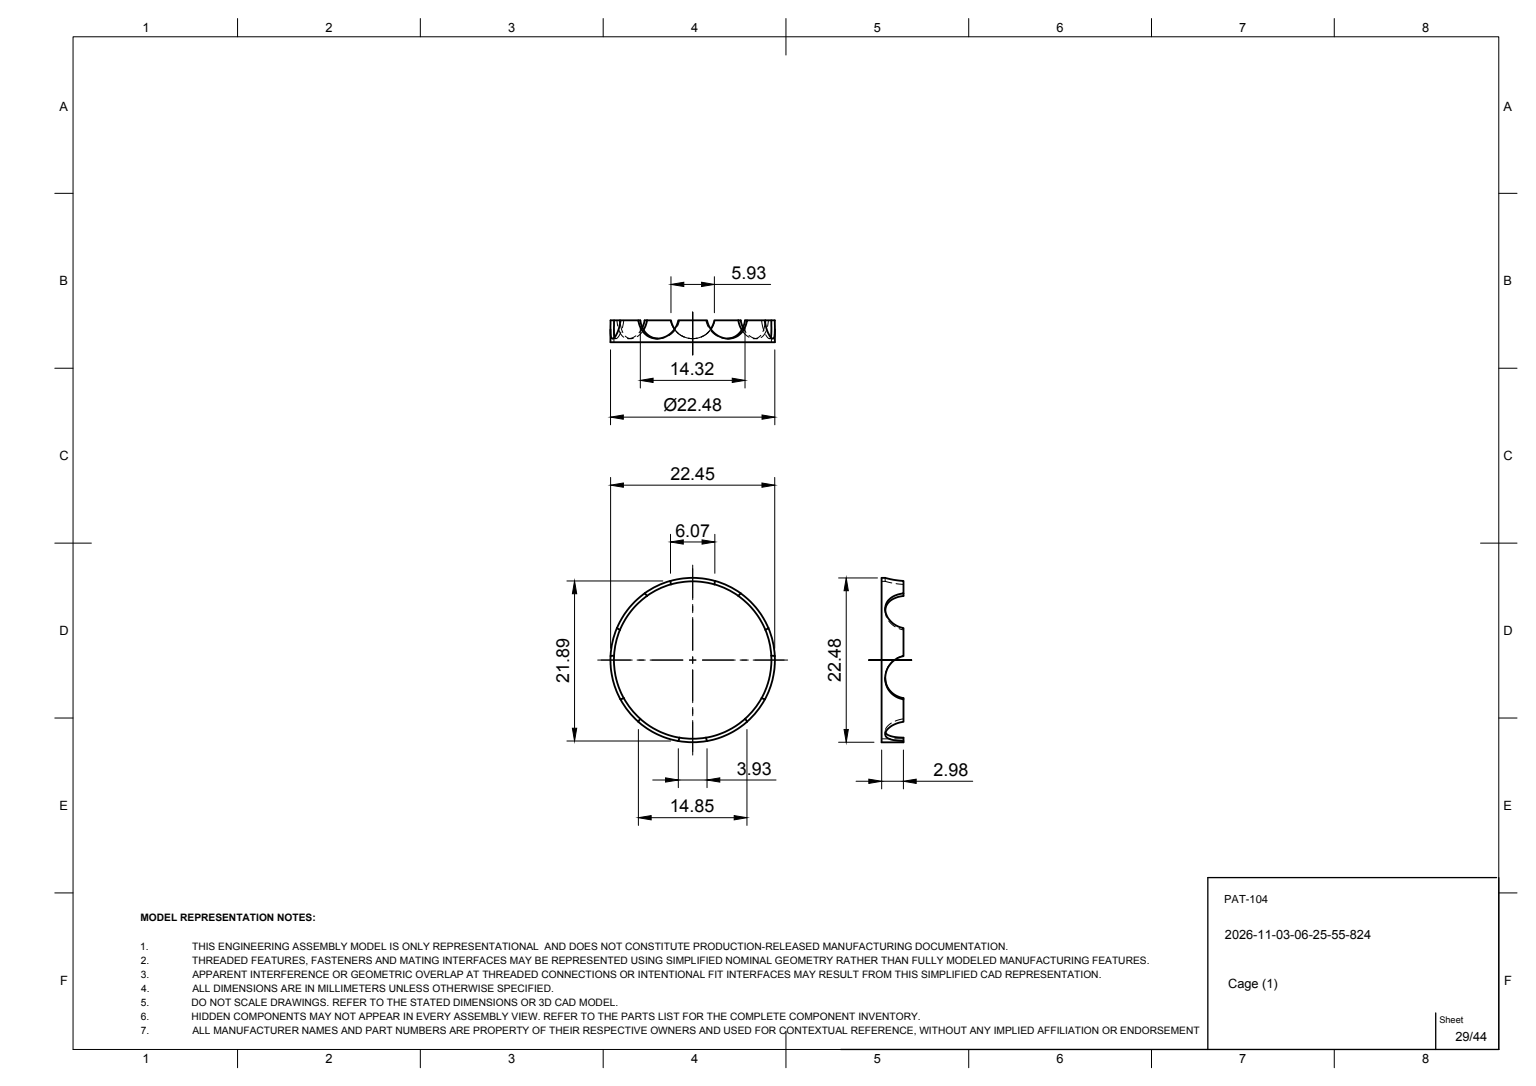
ISO-10303-21;
HEADER;
/* Generated by software containing ST-Developer
 * from STEP Tools, Inc. (www.steptools.com) 
 */

FILE_DESCRIPTION(
/* description */ ('Timing belt drive module 2 mm Pitch Timing 20T-40T'),

/* implementation_level */ '2;1');

FILE_NAME(
/* name */ 'Cage (1).step',
/* time_stamp */ '2026-10-28T03:25:12-07:00',
/* author */ (''),
/* organization */ (''),
/* preprocessor_version */ 'ST-DEVELOPER v20.2',
/* originating_system */ 'Autodesk Translation Framework v15.17.0.0',
/* authorisation */ '');

FILE_SCHEMA (('AUTOMOTIVE_DESIGN { 1 0 10303 214 3 1 1 }'));
ENDSEC;

DATA;
#10=MECHANICAL_DESIGN_GEOMETRIC_PRESENTATION_REPRESENTATION('',(#563),#17830);
#327=B_SPLINE_CURVE_WITH_KNOTS('',3,(#15464,#15465,#15466,#15467,#15468,
#15469,#15470,#15471,#15472,#15473,#15474,#15475,#15476,#15477,#15478,#15479,
#15480,#15481,#15482,#15483,#15484,#15485),.UNSPECIFIED.,.F.,.F.,(4,2,2,
2,2,2,2,2,2,2,4),(0.0591825211272536,0.157966726598481,0.236950089897721,
0.315933453196962,0.391576304923761,0.46721915665056,0.54286200837736,0.618504860104159,
0.697488223403399,0.77647158670264,0.875255792173867),.UNSPECIFIED.);
#328=B_SPLINE_CURVE_WITH_KNOTS('',3,(#15489,#15490,#15491,#15492,#15493,
#15494,#15495,#15496,#15497,#15498,#15499,#15500,#15501,#15502,#15503,#15504,
#15505,#15506,#15507,#15508,#15509,#15510),.UNSPECIFIED.,.F.,.F.,(4,2,2,
2,2,2,2,2,2,2,4),(0.0581119756758434,0.106553146291161,0.213106292582322,
0.30849933801665,0.386091982889075,0.4636846277615,0.541277272633925,0.61886991750635,
0.714262962940678,0.820816109231839,0.869257279847157),.UNSPECIFIED.);
#329=B_SPLINE_CURVE_WITH_KNOTS('',3,(#15516,#15517,#15518,#15519,#15520,
#15521,#15522,#15523,#15524,#15525,#15526,#15527,#15528,#15529,#15530,#15531,
#15532,#15533,#15534,#15535,#15536,#15537),.UNSPECIFIED.,.F.,.F.,(4,2,2,
2,2,2,2,2,2,2,4),(0.0581119756758434,0.106553146291161,0.213106292582322,
0.30849933801665,0.386091982889075,0.4636846277615,0.541277272633925,0.61886991750635,
0.714262962940679,0.820816109231839,0.869257279847157),.UNSPECIFIED.);
#330=B_SPLINE_CURVE_WITH_KNOTS('',3,(#15541,#15542,#15543,#15544,#15545,
#15546,#15547,#15548,#15549,#15550,#15551,#15552,#15553,#15554,#15555,#15556,
#15557,#15558,#15559,#15560,#15561,#15562),.UNSPECIFIED.,.F.,.F.,(4,2,2,
2,2,2,2,2,2,2,4),(0.0581119756758433,0.106553146291161,0.213106292582322,
0.308499338016649,0.386091982889075,0.4636846277615,0.541277272633925,0.61886991750635,
0.714262962940678,0.820816109231839,0.869257279847157),.UNSPECIFIED.);
#331=B_SPLINE_CURVE_WITH_KNOTS('',3,(#15571,#15572,#15573,#15574,#15575,
#15576,#15577,#15578,#15579,#15580,#15581,#15582,#15583,#15584,#15585,#15586,
#15587,#15588,#15589,#15590,#15591,#15592),.UNSPECIFIED.,.F.,.F.,(4,2,2,
2,2,2,2,2,2,2,4),(0.0581119756758433,0.106553146291161,0.213106292582322,
0.30849933801665,0.386091982889075,0.4636846277615,0.541277272633925,0.61886991750635,
0.714262962940678,0.820816109231839,0.869257279847157),.UNSPECIFIED.);
#332=B_SPLINE_CURVE_WITH_KNOTS('',3,(#15596,#15597,#15598,#15599,#15600,
#15601,#15602,#15603,#15604,#15605,#15606,#15607,#15608,#15609,#15610,#15611,
#15612,#15613,#15614,#15615,#15616,#15617),.UNSPECIFIED.,.F.,.F.,(4,2,2,
2,2,2,2,2,2,2,4),(0.0581119756758434,0.106553146291161,0.213106292582322,
0.30849933801665,0.386091982889075,0.4636846277615,0.541277272633925,0.61886991750635,
0.714262962940678,0.820816109231839,0.869257279847157),.UNSPECIFIED.);
#333=B_SPLINE_CURVE_WITH_KNOTS('',3,(#15621,#15622,#15623,#15624,#15625,
#15626,#15627,#15628,#15629,#15630,#15631,#15632,#15633,#15634,#15635,#15636,
#15637,#15638,#15639,#15640,#15641,#15642),.UNSPECIFIED.,.F.,.F.,(4,2,2,
2,2,2,2,2,2,2,4),(0.0581119756758434,0.106553146291161,0.213106292582322,
0.30849933801665,0.386091982889075,0.4636846277615,0.541277272633925,0.61886991750635,
0.714262962940678,0.820816109231839,0.869257279847157),.UNSPECIFIED.);
#334=B_SPLINE_CURVE_WITH_KNOTS('',3,(#15646,#15647,#15648,#15649,#15650,
#15651,#15652,#15653,#15654,#15655,#15656,#15657,#15658,#15659,#15660,#15661,
#15662,#15663,#15664,#15665,#15666,#15667),.UNSPECIFIED.,.F.,.F.,(4,2,2,
2,2,2,2,2,2,2,4),(0.0581119756758433,0.106553146291161,0.213106292582322,
0.30849933801665,0.386091982889075,0.4636846277615,0.541277272633925,0.61886991750635,
0.714262962940678,0.820816109231839,0.869257279847157),.UNSPECIFIED.);
#335=B_SPLINE_CURVE_WITH_KNOTS('',3,(#15675,#15676,#15677,#15678,#15679,
#15680,#15681,#15682,#15683,#15684,#15685,#15686,#15687,#15688,#15689,#15690,
#15691,#15692,#15693,#15694,#15695,#15696),.UNSPECIFIED.,.F.,.F.,(4,2,2,
2,2,2,2,2,2,2,4),(0.0591825211272536,0.157966726598481,0.236950089897721,
0.315933453196962,0.391576304923761,0.467219156650561,0.54286200837736,
0.618504860104159,0.697488223403399,0.77647158670264,0.875255792173867),
 .UNSPECIFIED.);
#336=B_SPLINE_CURVE_WITH_KNOTS('',3,(#15704,#15705,#15706,#15707,#15708,
#15709,#15710,#15711,#15712,#15713,#15714,#15715,#15716,#15717,#15718,#15719,
#15720,#15721,#15722,#15723,#15724,#15725),.UNSPECIFIED.,.F.,.F.,(4,2,2,
2,2,2,2,2,2,2,4),(0.0591825211272536,0.157966726598481,0.236950089897722,
0.315933453196962,0.391576304923761,0.467219156650561,0.54286200837736,
0.618504860104159,0.697488223403399,0.77647158670264,0.875255792173867),
 .UNSPECIFIED.);
#337=B_SPLINE_CURVE_WITH_KNOTS('',3,(#15735,#15736,#15737,#15738,#15739,
#15740,#15741,#15742,#15743,#15744,#15745,#15746,#15747,#15748,#15749,#15750,
#15751,#15752,#15753,#15754,#15755,#15756),.UNSPECIFIED.,.F.,.F.,(4,2,2,
2,2,2,2,2,2,2,4),(0.0591825211272536,0.157966726598481,0.236950089897721,
0.315933453196962,0.391576304923761,0.46721915665056,0.54286200837736,0.618504860104159,
0.697488223403399,0.77647158670264,0.875255792173867),.UNSPECIFIED.);
#338=B_SPLINE_CURVE_WITH_KNOTS('',3,(#15764,#15765,#15766,#15767,#15768,
#15769,#15770,#15771,#15772,#15773,#15774,#15775,#15776,#15777,#15778,#15779,
#15780,#15781,#15782,#15783,#15784,#15785),.UNSPECIFIED.,.F.,.F.,(4,2,2,
2,2,2,2,2,2,2,4),(0.0591825211272536,0.157966726598481,0.236950089897721,
0.315933453196962,0.391576304923761,0.46721915665056,0.542862008377359,
0.618504860104159,0.697488223403399,0.776471586702639,0.875255792173867),
 .UNSPECIFIED.);
#339=B_SPLINE_CURVE_WITH_KNOTS('',3,(#15793,#15794,#15795,#15796,#15797,
#15798,#15799,#15800,#15801,#15802,#15803,#15804,#15805,#15806,#15807,#15808,
#15809,#15810,#15811,#15812,#15813,#15814),.UNSPECIFIED.,.F.,.F.,(4,2,2,
2,2,2,2,2,2,2,4),(0.0591825211272536,0.157966726598481,0.236950089897721,
0.315933453196962,0.391576304923761,0.46721915665056,0.54286200837736,0.618504860104159,
0.697488223403399,0.77647158670264,0.875255792173867),.UNSPECIFIED.);
#340=B_SPLINE_CURVE_WITH_KNOTS('',3,(#15823,#15824,#15825,#15826,#15827,
#15828,#15829,#15830,#15831,#15832,#15833,#15834,#15835,#15836,#15837,#15838,
#15839,#15840,#15841,#15842,#15843,#15844),.UNSPECIFIED.,.F.,.F.,(4,2,2,
2,2,2,2,2,2,2,4),(0.0591825211272536,0.157966726598481,0.236950089897721,
0.315933453196962,0.391576304923761,0.46721915665056,0.542862008377359,
0.618504860104159,0.697488223403399,0.776471586702639,0.875255792173867),
 .UNSPECIFIED.);
#408=SPHERICAL_SURFACE('',#10097,0.309556);
#409=SPHERICAL_SURFACE('',#10113,0.309556);
#410=SPHERICAL_SURFACE('',#10118,0.309556);
#411=SPHERICAL_SURFACE('',#10124,0.309556);
#412=SPHERICAL_SURFACE('',#10129,0.309556);
#413=SPHERICAL_SURFACE('',#10134,0.309556);
#414=SPHERICAL_SURFACE('',#10142,0.309556);
#463=SHAPE_REPRESENTATION_RELATIONSHIP('SRR','None',#18035,#506);
#506=ADVANCED_BREP_SHAPE_REPRESENTATION('',(#620),#17810);
#563=STYLED_ITEM('',(#18317),#620);
#620=MANIFOLD_SOLID_BREP('Continuous crown cage',#9021);
#724=FACE_BOUND('',#1845,.T.);
#886=PLANE('',#10110);
#887=PLANE('',#10115);
#888=PLANE('',#10120);
#889=PLANE('',#10126);
#890=PLANE('',#10131);
#891=PLANE('',#10140);
#892=PLANE('',#10144);
#893=PLANE('',#10145);
#1221=FACE_OUTER_BOUND('',#1829,.T.);
#1222=FACE_OUTER_BOUND('',#1830,.T.);
#1223=FACE_OUTER_BOUND('',#1831,.T.);
#1224=FACE_OUTER_BOUND('',#1832,.T.);
#1225=FACE_OUTER_BOUND('',#1833,.T.);
#1226=FACE_OUTER_BOUND('',#1834,.T.);
#1227=FACE_OUTER_BOUND('',#1835,.T.);
#1228=FACE_OUTER_BOUND('',#1836,.T.);
#1229=FACE_OUTER_BOUND('',#1837,.T.);
#1230=FACE_OUTER_BOUND('',#1838,.T.);
#1231=FACE_OUTER_BOUND('',#1839,.T.);
#1232=FACE_OUTER_BOUND('',#1840,.T.);
#1233=FACE_OUTER_BOUND('',#1841,.T.);
#1234=FACE_OUTER_BOUND('',#1842,.T.);
#1235=FACE_OUTER_BOUND('',#1843,.T.);
#1236=FACE_OUTER_BOUND('',#1844,.T.);
#1237=FACE_OUTER_BOUND('',#1846,.T.);
#1829=EDGE_LOOP('',(#6901,#6902,#6903,#6904));
#1830=EDGE_LOOP('',(#6905,#6906,#6907,#6908,#6909,#6910,#6911,#6912,#6913,
#6914,#6915,#6916,#6917,#6918,#6919,#6920,#6921,#6922));
#1831=EDGE_LOOP('',(#6923,#6924,#6925,#6926));
#1832=EDGE_LOOP('',(#6927,#6928,#6929,#6930));
#1833=EDGE_LOOP('',(#6931,#6932,#6933,#6934));
#1834=EDGE_LOOP('',(#6935,#6936,#6937,#6938));
#1835=EDGE_LOOP('',(#6939,#6940,#6941,#6942,#6943,#6944));
#1836=EDGE_LOOP('',(#6945,#6946,#6947,#6948));
#1837=EDGE_LOOP('',(#6949,#6950,#6951,#6952));
#1838=EDGE_LOOP('',(#6953,#6954,#6955,#6956));
#1839=EDGE_LOOP('',(#6957,#6958,#6959,#6960));
#1840=EDGE_LOOP('',(#6961,#6962,#6963,#6964));
#1841=EDGE_LOOP('',(#6965,#6966,#6967,#6968,#6969,#6970,#6971,#6972,#6973,
#6974,#6975,#6976,#6977,#6978,#6979,#6980,#6981,#6982));
#1842=EDGE_LOOP('',(#6983,#6984,#6985,#6986));
#1843=EDGE_LOOP('',(#6987,#6988,#6989,#6990));
#1844=EDGE_LOOP('',(#6991));
#1845=EDGE_LOOP('',(#6992));
#1846=EDGE_LOOP('',(#6993,#6994,#6995,#6996));
#2427=CIRCLE('',#10098,0.303778037777585);
#2428=CIRCLE('',#10099,0.303778037777585);
#2429=CIRCLE('',#10101,1.123812);
#2430=CIRCLE('',#10102,1.123812);
#2431=CIRCLE('',#10103,1.123812);
#2432=CIRCLE('',#10104,1.123812);
#2433=CIRCLE('',#10105,1.123812);
#2434=CIRCLE('',#10106,1.123812);
#2435=CIRCLE('',#10107,1.123812);
#2436=CIRCLE('',#10108,1.123812);
#2437=CIRCLE('',#10109,1.123812);
#2438=CIRCLE('',#10111,1.076188);
#2439=CIRCLE('',#10112,0.303778037777585);
#2440=CIRCLE('',#10114,0.303778037777585);
#2441=CIRCLE('',#10116,1.076188);
#2442=CIRCLE('',#10117,0.303778037777585);
#2443=CIRCLE('',#10119,0.303778037777585);
#2444=CIRCLE('',#10121,1.076188);
#2445=CIRCLE('',#10122,1.076188);
#2446=CIRCLE('',#10123,0.303778037777585);
#2447=CIRCLE('',#10125,0.303778037777585);
#2448=CIRCLE('',#10127,1.076188);
#2449=CIRCLE('',#10128,0.303778037777585);
#2450=CIRCLE('',#10130,0.303778037777585);
#2451=CIRCLE('',#10132,1.076188);
#2452=CIRCLE('',#10133,0.303778037777585);
#2453=CIRCLE('',#10135,0.303778037777585);
#2454=CIRCLE('',#10137,1.076188);
#2455=CIRCLE('',#10138,1.076188);
#2456=CIRCLE('',#10139,1.076188);
#2457=CIRCLE('',#10141,0.303778037777585);
#2458=CIRCLE('',#10143,0.303778037777585);
#3049=LINE('',#15566,#3527);
#3050=LINE('',#15819,#3528);
#3527=VECTOR('',#12244,1.123812);
#3528=VECTOR('',#12313,1.076188);
#4138=VERTEX_POINT('',#15462);
#4139=VERTEX_POINT('',#15463);
#4140=VERTEX_POINT('',#15486);
#4141=VERTEX_POINT('',#15488);
#4142=VERTEX_POINT('',#15513);
#4143=VERTEX_POINT('',#15515);
#4144=VERTEX_POINT('',#15538);
#4145=VERTEX_POINT('',#15540);
#4146=VERTEX_POINT('',#15563);
#4147=VERTEX_POINT('',#15565);
#4148=VERTEX_POINT('',#15568);
#4149=VERTEX_POINT('',#15570);
#4150=VERTEX_POINT('',#15593);
#4151=VERTEX_POINT('',#15595);
#4152=VERTEX_POINT('',#15618);
#4153=VERTEX_POINT('',#15620);
#4154=VERTEX_POINT('',#15643);
#4155=VERTEX_POINT('',#15645);
#4156=VERTEX_POINT('',#15670);
#4157=VERTEX_POINT('',#15674);
#4158=VERTEX_POINT('',#15699);
#4159=VERTEX_POINT('',#15703);
#4160=VERTEX_POINT('',#15728);
#4161=VERTEX_POINT('',#15730);
#4162=VERTEX_POINT('',#15734);
#4163=VERTEX_POINT('',#15759);
#4164=VERTEX_POINT('',#15763);
#4165=VERTEX_POINT('',#15788);
#4166=VERTEX_POINT('',#15792);
#4167=VERTEX_POINT('',#15817);
#4168=VERTEX_POINT('',#15820);
#4169=VERTEX_POINT('',#15822);
#5133=EDGE_CURVE('',#4138,#4139,#327,.T.);
#5134=EDGE_CURVE('',#4140,#4138,#2427,.T.);
#5135=EDGE_CURVE('',#4141,#4140,#328,.T.);
#5136=EDGE_CURVE('',#4139,#4141,#2428,.T.);
#5137=EDGE_CURVE('',#4142,#4140,#2429,.T.);
#5138=EDGE_CURVE('',#4142,#4143,#329,.T.);
#5139=EDGE_CURVE('',#4144,#4143,#2430,.T.);
#5140=EDGE_CURVE('',#4144,#4145,#330,.T.);
#5141=EDGE_CURVE('',#4146,#4145,#2431,.T.);
#5142=EDGE_CURVE('',#4146,#4147,#3049,.T.);
#5143=EDGE_CURVE('',#4147,#4147,#2432,.T.);
#5144=EDGE_CURVE('',#4148,#4146,#2433,.T.);
#5145=EDGE_CURVE('',#4148,#4149,#331,.T.);
#5146=EDGE_CURVE('',#4150,#4149,#2434,.T.);
#5147=EDGE_CURVE('',#4150,#4151,#332,.T.);
#5148=EDGE_CURVE('',#4152,#4151,#2435,.T.);
#5149=EDGE_CURVE('',#4152,#4153,#333,.T.);
#5150=EDGE_CURVE('',#4154,#4153,#2436,.T.);
#5151=EDGE_CURVE('',#4154,#4155,#334,.T.);
#5152=EDGE_CURVE('',#4141,#4155,#2437,.T.);
#5153=EDGE_CURVE('',#4138,#4156,#2438,.T.);
#5154=EDGE_CURVE('',#4156,#4142,#2439,.T.);
#5155=EDGE_CURVE('',#4157,#4156,#335,.T.);
#5156=EDGE_CURVE('',#4143,#4157,#2440,.T.);
#5157=EDGE_CURVE('',#4157,#4158,#2441,.T.);
#5158=EDGE_CURVE('',#4158,#4144,#2442,.T.);
#5159=EDGE_CURVE('',#4159,#4158,#336,.T.);
#5160=EDGE_CURVE('',#4145,#4159,#2443,.T.);
#5161=EDGE_CURVE('',#4159,#4160,#2444,.T.);
#5162=EDGE_CURVE('',#4160,#4161,#2445,.T.);
#5163=EDGE_CURVE('',#4161,#4148,#2446,.T.);
#5164=EDGE_CURVE('',#4162,#4161,#337,.T.);
#5165=EDGE_CURVE('',#4149,#4162,#2447,.T.);
#5166=EDGE_CURVE('',#4162,#4163,#2448,.T.);
#5167=EDGE_CURVE('',#4163,#4150,#2449,.T.);
#5168=EDGE_CURVE('',#4164,#4163,#338,.T.);
#5169=EDGE_CURVE('',#4151,#4164,#2450,.T.);
#5170=EDGE_CURVE('',#4164,#4165,#2451,.T.);
#5171=EDGE_CURVE('',#4165,#4152,#2452,.T.);
#5172=EDGE_CURVE('',#4166,#4165,#339,.T.);
#5173=EDGE_CURVE('',#4153,#4166,#2453,.T.);
#5174=EDGE_CURVE('',#4167,#4167,#2454,.T.);
#5175=EDGE_CURVE('',#4167,#4160,#3050,.T.);
#5176=EDGE_CURVE('',#4168,#4139,#2455,.T.);
#5177=EDGE_CURVE('',#4168,#4169,#340,.T.);
#5178=EDGE_CURVE('',#4166,#4169,#2456,.T.);
#5179=EDGE_CURVE('',#4155,#4168,#2457,.T.);
#5180=EDGE_CURVE('',#4169,#4154,#2458,.T.);
#6901=ORIENTED_EDGE('',*,*,#5133,.F.);
#6902=ORIENTED_EDGE('',*,*,#5134,.F.);
#6903=ORIENTED_EDGE('',*,*,#5135,.F.);
#6904=ORIENTED_EDGE('',*,*,#5136,.F.);
#6905=ORIENTED_EDGE('',*,*,#5135,.T.);
#6906=ORIENTED_EDGE('',*,*,#5137,.F.);
#6907=ORIENTED_EDGE('',*,*,#5138,.T.);
#6908=ORIENTED_EDGE('',*,*,#5139,.F.);
#6909=ORIENTED_EDGE('',*,*,#5140,.T.);
#6910=ORIENTED_EDGE('',*,*,#5141,.F.);
#6911=ORIENTED_EDGE('',*,*,#5142,.T.);
#6912=ORIENTED_EDGE('',*,*,#5143,.F.);
#6913=ORIENTED_EDGE('',*,*,#5142,.F.);
#6914=ORIENTED_EDGE('',*,*,#5144,.F.);
#6915=ORIENTED_EDGE('',*,*,#5145,.T.);
#6916=ORIENTED_EDGE('',*,*,#5146,.F.);
#6917=ORIENTED_EDGE('',*,*,#5147,.T.);
#6918=ORIENTED_EDGE('',*,*,#5148,.F.);
#6919=ORIENTED_EDGE('',*,*,#5149,.T.);
#6920=ORIENTED_EDGE('',*,*,#5150,.F.);
#6921=ORIENTED_EDGE('',*,*,#5151,.T.);
#6922=ORIENTED_EDGE('',*,*,#5152,.F.);
#6923=ORIENTED_EDGE('',*,*,#5134,.T.);
#6924=ORIENTED_EDGE('',*,*,#5153,.T.);
#6925=ORIENTED_EDGE('',*,*,#5154,.T.);
#6926=ORIENTED_EDGE('',*,*,#5137,.T.);
#6927=ORIENTED_EDGE('',*,*,#5155,.F.);
#6928=ORIENTED_EDGE('',*,*,#5156,.F.);
#6929=ORIENTED_EDGE('',*,*,#5138,.F.);
#6930=ORIENTED_EDGE('',*,*,#5154,.F.);
#6931=ORIENTED_EDGE('',*,*,#5156,.T.);
#6932=ORIENTED_EDGE('',*,*,#5157,.T.);
#6933=ORIENTED_EDGE('',*,*,#5158,.T.);
#6934=ORIENTED_EDGE('',*,*,#5139,.T.);
#6935=ORIENTED_EDGE('',*,*,#5159,.F.);
#6936=ORIENTED_EDGE('',*,*,#5160,.F.);
#6937=ORIENTED_EDGE('',*,*,#5140,.F.);
#6938=ORIENTED_EDGE('',*,*,#5158,.F.);
#6939=ORIENTED_EDGE('',*,*,#5160,.T.);
#6940=ORIENTED_EDGE('',*,*,#5161,.T.);
#6941=ORIENTED_EDGE('',*,*,#5162,.T.);
#6942=ORIENTED_EDGE('',*,*,#5163,.T.);
#6943=ORIENTED_EDGE('',*,*,#5144,.T.);
#6944=ORIENTED_EDGE('',*,*,#5141,.T.);
#6945=ORIENTED_EDGE('',*,*,#5164,.F.);
#6946=ORIENTED_EDGE('',*,*,#5165,.F.);
#6947=ORIENTED_EDGE('',*,*,#5145,.F.);
#6948=ORIENTED_EDGE('',*,*,#5163,.F.);
#6949=ORIENTED_EDGE('',*,*,#5165,.T.);
#6950=ORIENTED_EDGE('',*,*,#5166,.T.);
#6951=ORIENTED_EDGE('',*,*,#5167,.T.);
#6952=ORIENTED_EDGE('',*,*,#5146,.T.);
#6953=ORIENTED_EDGE('',*,*,#5168,.F.);
#6954=ORIENTED_EDGE('',*,*,#5169,.F.);
#6955=ORIENTED_EDGE('',*,*,#5147,.F.);
#6956=ORIENTED_EDGE('',*,*,#5167,.F.);
#6957=ORIENTED_EDGE('',*,*,#5169,.T.);
#6958=ORIENTED_EDGE('',*,*,#5170,.T.);
#6959=ORIENTED_EDGE('',*,*,#5171,.T.);
#6960=ORIENTED_EDGE('',*,*,#5148,.T.);
#6961=ORIENTED_EDGE('',*,*,#5149,.F.);
#6962=ORIENTED_EDGE('',*,*,#5171,.F.);
#6963=ORIENTED_EDGE('',*,*,#5172,.F.);
#6964=ORIENTED_EDGE('',*,*,#5173,.F.);
#6965=ORIENTED_EDGE('',*,*,#5174,.F.);
#6966=ORIENTED_EDGE('',*,*,#5175,.T.);
#6967=ORIENTED_EDGE('',*,*,#5161,.F.);
#6968=ORIENTED_EDGE('',*,*,#5159,.T.);
#6969=ORIENTED_EDGE('',*,*,#5157,.F.);
#6970=ORIENTED_EDGE('',*,*,#5155,.T.);
#6971=ORIENTED_EDGE('',*,*,#5153,.F.);
#6972=ORIENTED_EDGE('',*,*,#5133,.T.);
#6973=ORIENTED_EDGE('',*,*,#5176,.F.);
#6974=ORIENTED_EDGE('',*,*,#5177,.T.);
#6975=ORIENTED_EDGE('',*,*,#5178,.F.);
#6976=ORIENTED_EDGE('',*,*,#5172,.T.);
#6977=ORIENTED_EDGE('',*,*,#5170,.F.);
#6978=ORIENTED_EDGE('',*,*,#5168,.T.);
#6979=ORIENTED_EDGE('',*,*,#5166,.F.);
#6980=ORIENTED_EDGE('',*,*,#5164,.T.);
#6981=ORIENTED_EDGE('',*,*,#5162,.F.);
#6982=ORIENTED_EDGE('',*,*,#5175,.F.);
#6983=ORIENTED_EDGE('',*,*,#5136,.T.);
#6984=ORIENTED_EDGE('',*,*,#5152,.T.);
#6985=ORIENTED_EDGE('',*,*,#5179,.T.);
#6986=ORIENTED_EDGE('',*,*,#5176,.T.);
#6987=ORIENTED_EDGE('',*,*,#5151,.F.);
#6988=ORIENTED_EDGE('',*,*,#5180,.F.);
#6989=ORIENTED_EDGE('',*,*,#5177,.F.);
#6990=ORIENTED_EDGE('',*,*,#5179,.F.);
#6991=ORIENTED_EDGE('',*,*,#5143,.T.);
#6992=ORIENTED_EDGE('',*,*,#5174,.T.);
#6993=ORIENTED_EDGE('',*,*,#5173,.T.);
#6994=ORIENTED_EDGE('',*,*,#5178,.T.);
#6995=ORIENTED_EDGE('',*,*,#5180,.T.);
#6996=ORIENTED_EDGE('',*,*,#5150,.T.);
#8288=CYLINDRICAL_SURFACE('',#10100,1.123812);
#8289=CYLINDRICAL_SURFACE('',#10136,1.076188);
#8719=ADVANCED_FACE('',(#1221),#408,.F.);
#8720=ADVANCED_FACE('',(#1222),#8288,.T.);
#8721=ADVANCED_FACE('',(#1223),#886,.T.);
#8722=ADVANCED_FACE('',(#1224),#409,.F.);
#8723=ADVANCED_FACE('',(#1225),#887,.T.);
#8724=ADVANCED_FACE('',(#1226),#410,.F.);
#8725=ADVANCED_FACE('',(#1227),#888,.T.);
#8726=ADVANCED_FACE('',(#1228),#411,.F.);
#8727=ADVANCED_FACE('',(#1229),#889,.T.);
#8728=ADVANCED_FACE('',(#1230),#412,.F.);
#8729=ADVANCED_FACE('',(#1231),#890,.T.);
#8730=ADVANCED_FACE('',(#1232),#413,.F.);
#8731=ADVANCED_FACE('',(#1233),#8289,.F.);
#8732=ADVANCED_FACE('',(#1234),#891,.T.);
#8733=ADVANCED_FACE('',(#1235),#414,.F.);
#8734=ADVANCED_FACE('',(#1236,#724),#892,.T.);
#8735=ADVANCED_FACE('',(#1237),#893,.T.);
#9021=CLOSED_SHELL('',(#8719,#8720,#8721,#8722,#8723,#8724,#8725,#8726,
#8727,#8728,#8729,#8730,#8731,#8732,#8733,#8734,#8735));
#10096=AXIS2_PLACEMENT_3D('',#15460,#12228,#12229);
#10097=AXIS2_PLACEMENT_3D('',#15461,#12230,#12231);
#10098=AXIS2_PLACEMENT_3D('',#15487,#12232,#12233);
#10099=AXIS2_PLACEMENT_3D('',#15511,#12234,#12235);
#10100=AXIS2_PLACEMENT_3D('',#15512,#12236,#12237);
#10101=AXIS2_PLACEMENT_3D('',#15514,#12238,#12239);
#10102=AXIS2_PLACEMENT_3D('',#15539,#12240,#12241);
#10103=AXIS2_PLACEMENT_3D('',#15564,#12242,#12243);
#10104=AXIS2_PLACEMENT_3D('',#15567,#12245,#12246);
#10105=AXIS2_PLACEMENT_3D('',#15569,#12247,#12248);
#10106=AXIS2_PLACEMENT_3D('',#15594,#12249,#12250);
#10107=AXIS2_PLACEMENT_3D('',#15619,#12251,#12252);
#10108=AXIS2_PLACEMENT_3D('',#15644,#12253,#12254);
#10109=AXIS2_PLACEMENT_3D('',#15668,#12255,#12256);
#10110=AXIS2_PLACEMENT_3D('',#15669,#12257,#12258);
#10111=AXIS2_PLACEMENT_3D('',#15671,#12259,#12260);
#10112=AXIS2_PLACEMENT_3D('',#15672,#12261,#12262);
#10113=AXIS2_PLACEMENT_3D('',#15673,#12263,#12264);
#10114=AXIS2_PLACEMENT_3D('',#15697,#12265,#12266);
#10115=AXIS2_PLACEMENT_3D('',#15698,#12267,#12268);
#10116=AXIS2_PLACEMENT_3D('',#15700,#12269,#12270);
#10117=AXIS2_PLACEMENT_3D('',#15701,#12271,#12272);
#10118=AXIS2_PLACEMENT_3D('',#15702,#12273,#12274);
#10119=AXIS2_PLACEMENT_3D('',#15726,#12275,#12276);
#10120=AXIS2_PLACEMENT_3D('',#15727,#12277,#12278);
#10121=AXIS2_PLACEMENT_3D('',#15729,#12279,#12280);
#10122=AXIS2_PLACEMENT_3D('',#15731,#12281,#12282);
#10123=AXIS2_PLACEMENT_3D('',#15732,#12283,#12284);
#10124=AXIS2_PLACEMENT_3D('',#15733,#12285,#12286);
#10125=AXIS2_PLACEMENT_3D('',#15757,#12287,#12288);
#10126=AXIS2_PLACEMENT_3D('',#15758,#12289,#12290);
#10127=AXIS2_PLACEMENT_3D('',#15760,#12291,#12292);
#10128=AXIS2_PLACEMENT_3D('',#15761,#12293,#12294);
#10129=AXIS2_PLACEMENT_3D('',#15762,#12295,#12296);
#10130=AXIS2_PLACEMENT_3D('',#15786,#12297,#12298);
#10131=AXIS2_PLACEMENT_3D('',#15787,#12299,#12300);
#10132=AXIS2_PLACEMENT_3D('',#15789,#12301,#12302);
#10133=AXIS2_PLACEMENT_3D('',#15790,#12303,#12304);
#10134=AXIS2_PLACEMENT_3D('',#15791,#12305,#12306);
#10135=AXIS2_PLACEMENT_3D('',#15815,#12307,#12308);
#10136=AXIS2_PLACEMENT_3D('',#15816,#12309,#12310);
#10137=AXIS2_PLACEMENT_3D('',#15818,#12311,#12312);
#10138=AXIS2_PLACEMENT_3D('',#15821,#12314,#12315);
#10139=AXIS2_PLACEMENT_3D('',#15845,#12316,#12317);
#10140=AXIS2_PLACEMENT_3D('',#15846,#12318,#12319);
#10141=AXIS2_PLACEMENT_3D('',#15847,#12320,#12321);
#10142=AXIS2_PLACEMENT_3D('',#15848,#12322,#12323);
#10143=AXIS2_PLACEMENT_3D('',#15849,#12324,#12325);
#10144=AXIS2_PLACEMENT_3D('',#15850,#12326,#12327);
#10145=AXIS2_PLACEMENT_3D('',#15851,#12328,#12329);
#12228=DIRECTION('axis',(0.,0.,1.));
#12229=DIRECTION('refdir',(1.,0.,0.));
#12230=DIRECTION('center_axis',(0.,0.,1.));
#12231=DIRECTION('ref_axis',(1.,0.,0.));
#12232=DIRECTION('center_axis',(0.,-1.,0.));
#12233=DIRECTION('ref_axis',(0.,0.,-1.));
#12234=DIRECTION('center_axis',(0.,-1.,0.));
#12235=DIRECTION('ref_axis',(0.,0.,-1.));
#12236=DIRECTION('center_axis',(0.,1.,0.));
#12237=DIRECTION('ref_axis',(1.,0.,0.));
#12238=DIRECTION('center_axis',(0.,1.,0.));
#12239=DIRECTION('ref_axis',(1.,0.,0.));
#12240=DIRECTION('center_axis',(0.,1.,0.));
#12241=DIRECTION('ref_axis',(1.,0.,0.));
#12242=DIRECTION('center_axis',(0.,1.,0.));
#12243=DIRECTION('ref_axis',(1.,0.,0.));
#12244=DIRECTION('',(0.,-1.,0.));
#12245=DIRECTION('center_axis',(0.,-1.,0.));
#12246=DIRECTION('ref_axis',(1.,0.,0.));
#12247=DIRECTION('center_axis',(0.,1.,0.));
#12248=DIRECTION('ref_axis',(1.,0.,0.));
#12249=DIRECTION('center_axis',(0.,1.,0.));
#12250=DIRECTION('ref_axis',(1.,0.,0.));
#12251=DIRECTION('center_axis',(0.,1.,0.));
#12252=DIRECTION('ref_axis',(1.,0.,0.));
#12253=DIRECTION('center_axis',(0.,1.,0.));
#12254=DIRECTION('ref_axis',(1.,0.,0.));
#12255=DIRECTION('center_axis',(0.,1.,0.));
#12256=DIRECTION('ref_axis',(1.,0.,0.));
#12257=DIRECTION('center_axis',(0.,1.,0.));
#12258=DIRECTION('ref_axis',(1.,0.,0.));
#12259=DIRECTION('center_axis',(0.,-1.,0.));
#12260=DIRECTION('ref_axis',(1.,0.,0.));
#12261=DIRECTION('center_axis',(0.,-1.,0.));
#12262=DIRECTION('ref_axis',(0.,0.,-1.));
#12263=DIRECTION('center_axis',(8.96625347776458E-17,0.,1.));
#12264=DIRECTION('ref_axis',(1.,0.,0.));
#12265=DIRECTION('center_axis',(0.,-1.,0.));
#12266=DIRECTION('ref_axis',(0.,0.,-1.));
#12267=DIRECTION('center_axis',(0.,1.,0.));
#12268=DIRECTION('ref_axis',(1.,0.,0.));
#12269=DIRECTION('center_axis',(0.,-1.,0.));
#12270=DIRECTION('ref_axis',(1.,0.,0.));
#12271=DIRECTION('center_axis',(0.,-1.,0.));
#12272=DIRECTION('ref_axis',(0.,0.,-1.));
#12273=DIRECTION('center_axis',(0.,0.,1.));
#12274=DIRECTION('ref_axis',(1.,0.,0.));
#12275=DIRECTION('center_axis',(0.,-1.,0.));
#12276=DIRECTION('ref_axis',(0.,0.,-1.));
#12277=DIRECTION('center_axis',(0.,1.,0.));
#12278=DIRECTION('ref_axis',(1.,0.,0.));
#12279=DIRECTION('center_axis',(0.,-1.,0.));
#12280=DIRECTION('ref_axis',(1.,0.,0.));
#12281=DIRECTION('center_axis',(0.,-1.,0.));
#12282=DIRECTION('ref_axis',(1.,0.,0.));
#12283=DIRECTION('center_axis',(0.,-1.,0.));
#12284=DIRECTION('ref_axis',(0.,0.,-1.));
#12285=DIRECTION('center_axis',(0.,0.,1.));
#12286=DIRECTION('ref_axis',(1.,0.,0.));
#12287=DIRECTION('center_axis',(0.,-1.,0.));
#12288=DIRECTION('ref_axis',(0.,0.,-1.));
#12289=DIRECTION('center_axis',(0.,1.,0.));
#12290=DIRECTION('ref_axis',(1.,0.,0.));
#12291=DIRECTION('center_axis',(0.,-1.,0.));
#12292=DIRECTION('ref_axis',(1.,0.,0.));
#12293=DIRECTION('center_axis',(0.,-1.,0.));
#12294=DIRECTION('ref_axis',(0.,0.,-1.));
#12295=DIRECTION('center_axis',(8.96625347776458E-17,0.,1.));
#12296=DIRECTION('ref_axis',(1.,0.,0.));
#12297=DIRECTION('center_axis',(0.,-1.,0.));
#12298=DIRECTION('ref_axis',(0.,0.,-1.));
#12299=DIRECTION('center_axis',(0.,1.,0.));
#12300=DIRECTION('ref_axis',(1.,0.,0.));
#12301=DIRECTION('center_axis',(0.,-1.,0.));
#12302=DIRECTION('ref_axis',(1.,0.,0.));
#12303=DIRECTION('center_axis',(0.,-1.,0.));
#12304=DIRECTION('ref_axis',(0.,0.,-1.));
#12305=DIRECTION('center_axis',(0.,0.,1.));
#12306=DIRECTION('ref_axis',(1.,0.,0.));
#12307=DIRECTION('center_axis',(0.,-1.,0.));
#12308=DIRECTION('ref_axis',(0.,0.,-1.));
#12309=DIRECTION('center_axis',(0.,1.,0.));
#12310=DIRECTION('ref_axis',(1.,0.,0.));
#12311=DIRECTION('center_axis',(0.,1.,0.));
#12312=DIRECTION('ref_axis',(1.,0.,0.));
#12313=DIRECTION('',(0.,1.,0.));
#12314=DIRECTION('center_axis',(0.,-1.,0.));
#12315=DIRECTION('ref_axis',(1.,0.,0.));
#12316=DIRECTION('center_axis',(0.,-1.,0.));
#12317=DIRECTION('ref_axis',(1.,0.,0.));
#12318=DIRECTION('center_axis',(0.,1.,0.));
#12319=DIRECTION('ref_axis',(1.,0.,0.));
#12320=DIRECTION('center_axis',(0.,-1.,0.));
#12321=DIRECTION('ref_axis',(0.,0.,-1.));
#12322=DIRECTION('center_axis',(0.,0.,1.));
#12323=DIRECTION('ref_axis',(1.,0.,0.));
#12324=DIRECTION('center_axis',(0.,-1.,0.));
#12325=DIRECTION('ref_axis',(0.,0.,-1.));
#12326=DIRECTION('center_axis',(0.,-1.,0.));
#12327=DIRECTION('ref_axis',(-1.,0.,0.));
#12328=DIRECTION('center_axis',(0.,1.,0.));
#12329=DIRECTION('ref_axis',(1.,0.,0.));
#15460=CARTESIAN_POINT('',(0.,0.,0.));
#15461=CARTESIAN_POINT('Origin',(0.685838782044607,0.,0.860014630714833));
#15462=CARTESIAN_POINT('',(0.413083465285518,-0.05953,0.993751811093549));
#15463=CARTESIAN_POINT('',(0.876916659919095,-0.05953,0.623857181492959));
#15464=CARTESIAN_POINT('Ctrl Pts',(0.413083465285518,-0.05953,0.993751811093549));
#15465=CARTESIAN_POINT('Ctrl Pts',(0.419070565453383,-0.0925528133349865,
0.991263089003441));
#15466=CARTESIAN_POINT('Ctrl Pts',(0.430199341854858,-0.124911173756694,
0.986608710139579));
#15467=CARTESIAN_POINT('Ctrl Pts',(0.457978755888596,-0.177924977804098,
0.973971221090534));
#15468=CARTESIAN_POINT('Ctrl Pts',(0.473077587363685,-0.199697230012983,
0.966820759530997));
#15469=CARTESIAN_POINT('Ctrl Pts',(0.507057380724533,-0.237895043532788,
0.949440676105255));
#15470=CARTESIAN_POINT('Ctrl Pts',(0.525933334162555,-0.254319232363049,
0.939198248544428));
#15471=CARTESIAN_POINT('Ctrl Pts',(0.564362943424238,-0.28018331644634,
0.916597376014514));
#15472=CARTESIAN_POINT('Ctrl Pts',(0.585840553788742,-0.29104845371857,
0.903141581680914));
#15473=CARTESIAN_POINT('Ctrl Pts',(0.629305439856167,-0.30527573347708,
0.873412008702649));
#15474=CARTESIAN_POINT('Ctrl Pts',(0.651278921914856,-0.308638795020976,
0.857118508332695));
#15475=CARTESIAN_POINT('Ctrl Pts',(0.690705563850638,-0.308638795020976,
0.825676810575914));
#15476=CARTESIAN_POINT('Ctrl Pts',(0.711480111898423,-0.30527573347708,
0.807879894508811));
#15477=CARTESIAN_POINT('Ctrl Pts',(0.750136149454208,-0.29104845371857,
0.772120216227122));
#15478=CARTESIAN_POINT('Ctrl Pts',(0.768033796848072,-0.28018331644634,
0.754175290318038));
#15479=CARTESIAN_POINT('Ctrl Pts',(0.798619410861634,-0.254319232363049,
0.721738358858166));
#15480=CARTESIAN_POINT('Ctrl Pts',(0.812805334167529,-0.237895043532788,
0.705614819529209));
#15481=CARTESIAN_POINT('Ctrl Pts',(0.837310877969633,-0.199697230012983,
0.676354402927683));
#15482=CARTESIAN_POINT('Ctrl Pts',(0.847641868610495,-0.177924977804098,
0.663225258065736));
#15483=CARTESIAN_POINT('Ctrl Pts',(0.866144010579847,-0.124911173756694,
0.638954437806245));
#15484=CARTESIAN_POINT('Ctrl Pts',(0.873158080166742,-0.0925528133349865,
0.62914037979579));
#15485=CARTESIAN_POINT('Ctrl Pts',(0.876916659919095,-0.05953,0.623857181492959));
#15486=CARTESIAN_POINT('',(0.437601487681057,-0.05953,1.03511272300331));
#15487=CARTESIAN_POINT('Origin',(0.685838782044607,-0.05953,0.860014630714833));
#15488=CARTESIAN_POINT('',(0.911784794170997,-0.05953,0.656964154625313));
#15489=CARTESIAN_POINT('Ctrl Pts',(0.911784794170998,-0.0595300000000001,
0.656964154625312));
#15490=CARTESIAN_POINT('Ctrl Pts',(0.909827729890942,-0.0762225747374255,
0.659680317203144));
#15491=CARTESIAN_POINT('Ctrl Pts',(0.907004864562642,-0.0928409665394228,
0.663576540841106));
#15492=CARTESIAN_POINT('Ctrl Pts',(0.895234408667242,-0.144299303100741,
0.679480524217551));
#15493=CARTESIAN_POINT('Ctrl Pts',(0.882797231409153,-0.177024326825049,
0.695831250979106));
#15494=CARTESIAN_POINT('Ctrl Pts',(0.854332839576145,-0.227269801620064,
0.73042219438957));
#15495=CARTESIAN_POINT('Ctrl Pts',(0.834863020612702,-0.251265615809407,
0.752807465209441));
#15496=CARTESIAN_POINT('Ctrl Pts',(0.800439809856111,-0.279889827963178,
0.789147407129766));
#15497=CARTESIAN_POINT('Ctrl Pts',(0.781998747691871,-0.290879136862659,
0.80756613568454));
#15498=CARTESIAN_POINT('Ctrl Pts',(0.742239891936898,-0.305251990234487,
0.844254137480382));
#15499=CARTESIAN_POINT('Ctrl Pts',(0.720906778729541,-0.308638795020976,
0.862505527716294));
#15500=CARTESIAN_POINT('Ctrl Pts',(0.680463863683392,-0.308638795020976,
0.894757676234429));
#15501=CARTESIAN_POINT('Ctrl Pts',(0.657923009631182,-0.305251990234488,
0.91149460735272));
#15502=CARTESIAN_POINT('Ctrl Pts',(0.613307674922609,-0.290879136862659,
0.942092777160053));
#15503=CARTESIAN_POINT('Ctrl Pts',(0.591247219971725,-0.279889827963178,
0.955972930713954));
#15504=CARTESIAN_POINT('Ctrl Pts',(0.548158511259202,-0.251265615809407,
0.981446681891443));
#15505=CARTESIAN_POINT('Ctrl Pts',(0.522002043615455,-0.227269801620063,
0.995447160474328));
#15506=CARTESIAN_POINT('Ctrl Pts',(0.481944444320713,-0.177024326825049,
1.01550068154148));
#15507=CARTESIAN_POINT('Ctrl Pts',(0.463236132117164,-0.14429930310074,
1.0239876538093));
#15508=CARTESIAN_POINT('Ctrl Pts',(0.445111721969657,-0.0928409665394226,
1.03192403056628));
#15509=CARTESIAN_POINT('Ctrl Pts',(0.440685038163619,-0.0762225747374254,
1.03380912944435));
#15510=CARTESIAN_POINT('Ctrl Pts',(0.437601487681056,-0.05953,1.03511272300331));
#15511=CARTESIAN_POINT('Origin',(0.685838782044607,-0.05953,0.860014630714833));
#15512=CARTESIAN_POINT('Origin',(0.,-0.208355,0.));
#15513=CARTESIAN_POINT('',(0.0548532617164168,-0.05953,1.12247250791415));
#15514=CARTESIAN_POINT('Origin',(0.,-0.05953,0.));
#15515=CARTESIAN_POINT('',(-0.536443649899848,-0.05953,0.987512846410683));
#15516=CARTESIAN_POINT('Ctrl Pts',(0.0548532617164173,-0.0595300000000001,
1.12247250791414));
#15517=CARTESIAN_POINT('Ctrl Pts',(0.05150947068137,-0.0762225747374254,
1.12263591311425));
#15518=CARTESIAN_POINT('Ctrl Pts',(0.0467032526342597,-0.0928409665394227,
1.12285816383385));
#15519=CARTESIAN_POINT('Ctrl Pts',(0.0269302585198975,-0.144299303100741,
1.12357162229597));
#15520=CARTESIAN_POINT('Ctrl Pts',(0.006392292392153,-0.177024326825049,
1.12404235695137));
#15521=CARTESIAN_POINT('Ctrl Pts',(-0.0383992541984087,-0.227269801620063,
1.12335509974011));
#15522=CARTESIAN_POINT('Ctrl Pts',(-0.0680399972366993,-0.251265615809407,
1.12208997038458));
#15523=CARTESIAN_POINT('Ctrl Pts',(-0.117914228755037,-0.279889827963178,
1.1178344036749));
#15524=CARTESIAN_POINT('Ctrl Pts',(-0.14381238480104,-0.290879136862659,
1.11490049012186));
#15525=CARTESIAN_POINT('Ctrl Pts',(-0.19728546073067,-0.305251990234488,
1.10669035995599));
#15526=CARTESIAN_POINT('Ctrl Pts',(-0.224855950742601,-0.308638795020976,
1.10139101611326));
#15527=CARTESIAN_POINT('Ctrl Pts',(-0.275287440920027,-0.308638795020976,
1.0898803575765));
#15528=CARTESIAN_POINT('Ctrl Pts',(-0.302426893214945,-0.305251990234488,
1.08269251410343));
#15529=CARTESIAN_POINT('Ctrl Pts',(-0.35416671187353,-0.290879136862659,
1.06688848765783));
#15530=CARTESIAN_POINT('Ctrl Pts',(-0.3787731215897,-0.279889827963178,
1.05829506364875));
#15531=CARTESIAN_POINT('Ctrl Pts',(-0.425554672694338,-0.251265615809407,
1.04048957871266));
#15532=CARTESIAN_POINT('Ctrl Pts',(-0.452808978448581,-0.227269801620063,
1.02876878445619));
#15533=CARTESIAN_POINT('Ctrl Pts',(-0.493462957200432,-0.177024326825049,
1.0099536580922));
#15534=CARTESIAN_POINT('Ctrl Pts',(-0.511762781179148,-0.14429930310074,
1.00061845128527));
#15535=CARTESIAN_POINT('Ctrl Pts',(-0.529268075276157,-0.0928409665394226,
0.991396466802468));
#15536=CARTESIAN_POINT('Ctrl Pts',(-0.533501897135713,-0.0762225747374254,
0.989110885965947));
#15537=CARTESIAN_POINT('Ctrl Pts',(-0.536443649899848,-0.0595300000000001,
0.987512846410683));
#15538=CARTESIAN_POINT('',(-0.843383895613249,-0.05953,0.742736168477219));
#15539=CARTESIAN_POINT('Origin',(0.,-0.05953,0.));
#15540=CARTESIAN_POINT('',(-1.10653577764992,-0.05953,0.196295654879792));
#15541=CARTESIAN_POINT('Ctrl Pts',(-0.843383895613249,-0.0595300000000001,
0.742736168477219));
#15542=CARTESIAN_POINT('Ctrl Pts',(-0.84559647055299,-0.0762225747374255,
0.740223768851062));
#15543=CARTESIAN_POINT('Ctrl Pts',(-0.848766861100456,-0.0928409665394227,
0.736604687327351));
#15544=CARTESIAN_POINT('Ctrl Pts',(-0.861652925570091,-0.144299303100741,
0.721590372101268));
#15545=CARTESIAN_POINT('Ctrl Pts',(-0.87482617317514,-0.177024326825049,
0.705826641853758));
#15546=CARTESIAN_POINT('Ctrl Pts',(-0.902215926359523,-0.227269801620063,
0.670378702718353));
#15547=CARTESIAN_POINT('Ctrl Pts',(-0.919707509403859,-0.251265615809407,
0.646415841396062));
#15548=CARTESIAN_POINT('Ctrl Pts',(-0.947476448101718,-0.279889827963178,
0.604769294586516));
#15549=CARTESIAN_POINT('Ctrl Pts',(-0.961329858300736,-0.290879136862659,
0.582692035672022));
#15550=CARTESIAN_POINT('Ctrl Pts',(-0.988250837578047,-0.305251990234488,
0.535766169015486));
#15551=CARTESIAN_POINT('Ctrl Pts',(-1.00129756308006,-0.308638795020976,
0.510906605094603));
#15552=CARTESIAN_POINT('Ctrl Pts',(-1.02374168767024,-0.308638795020976,
0.46430090015576));
#15553=CARTESIAN_POINT('Ctrl Pts',(-1.03504317708586,-0.305251990234488,
0.438600874831839));
#15554=CARTESIAN_POINT('Ctrl Pts',(-1.05494634094458,-0.290879136862659,
0.388295406390235));
#15555=CARTESIAN_POINT('Ctrl Pts',(-1.06356957703048,-0.279889827963178,
0.363699428370917));
#15556=CARTESIAN_POINT('Ctrl Pts',(-1.0788165083757,-0.251265615809407,
0.316022600643821));
#15557=CARTESIAN_POINT('Ctrl Pts',(-1.08664560412098,-0.227269801620063,
0.287406530683752));
#15558=CARTESIAN_POINT('Ctrl Pts',(-1.09728268713976,-0.177024326825049,
0.243890930799337));
#15559=CARTESIAN_POINT('Ctrl Pts',(-1.10139388218929,-0.144299303100741,
0.22376314604679));
#15560=CARTESIAN_POINT('Ctrl Pts',(-1.10509821673782,-0.0928409665394227,
0.204327142733961));
#15561=CARTESIAN_POINT('Ctrl Pts',(-1.10595102243643,-0.0762225747374254,
0.199591971170104));
#15562=CARTESIAN_POINT('Ctrl Pts',(-1.10653577764992,-0.0595300000000001,
0.196295654879792));
#15563=CARTESIAN_POINT('',(-1.123812,-0.05953,1.37627276864339E-16));
#15564=CARTESIAN_POINT('Origin',(0.,-0.05953,0.));
#15565=CARTESIAN_POINT('',(-1.123812,-0.35718,1.37627276864339E-16));
#15566=CARTESIAN_POINT('',(-1.123812,-0.208355,1.37627276864339E-16));
#15567=CARTESIAN_POINT('Origin',(0.,-0.35718,0.));
#15568=CARTESIAN_POINT('',(-1.10653577764992,-0.05953,-0.196295654879793));
#15569=CARTESIAN_POINT('Origin',(0.,-0.05953,0.));
#15570=CARTESIAN_POINT('',(-0.843383895613249,-0.05953,-0.742736168477219));
#15571=CARTESIAN_POINT('Ctrl Pts',(-1.10653577764992,-0.0595300000000001,
-0.196295654879792));
#15572=CARTESIAN_POINT('Ctrl Pts',(-1.10595102243643,-0.0762225747374255,
-0.199591971170104));
#15573=CARTESIAN_POINT('Ctrl Pts',(-1.10509821673782,-0.0928409665394228,
-0.204327142733962));
#15574=CARTESIAN_POINT('Ctrl Pts',(-1.10139388218929,-0.144299303100741,
-0.22376314604679));
#15575=CARTESIAN_POINT('Ctrl Pts',(-1.09728268713976,-0.177024326825049,
-0.243890930799338));
#15576=CARTESIAN_POINT('Ctrl Pts',(-1.08664560412098,-0.227269801620063,
-0.287406530683753));
#15577=CARTESIAN_POINT('Ctrl Pts',(-1.0788165083757,-0.251265615809407,
-0.316022600643821));
#15578=CARTESIAN_POINT('Ctrl Pts',(-1.06356957703048,-0.279889827963178,
-0.363699428370918));
#15579=CARTESIAN_POINT('Ctrl Pts',(-1.05494634094458,-0.290879136862659,
-0.388295406390235));
#15580=CARTESIAN_POINT('Ctrl Pts',(-1.03504317708586,-0.305251990234488,
-0.438600874831839));
#15581=CARTESIAN_POINT('Ctrl Pts',(-1.02374168767024,-0.308638795020976,
-0.46430090015576));
#15582=CARTESIAN_POINT('Ctrl Pts',(-1.00129756308006,-0.308638795020976,
-0.510906605094603));
#15583=CARTESIAN_POINT('Ctrl Pts',(-0.988250837578047,-0.305251990234488,
-0.535766169015486));
#15584=CARTESIAN_POINT('Ctrl Pts',(-0.961329858300736,-0.290879136862659,
-0.582692035672022));
#15585=CARTESIAN_POINT('Ctrl Pts',(-0.947476448101718,-0.279889827963178,
-0.604769294586516));
#15586=CARTESIAN_POINT('Ctrl Pts',(-0.919707509403859,-0.251265615809407,
-0.646415841396062));
#15587=CARTESIAN_POINT('Ctrl Pts',(-0.902215926359523,-0.227269801620064,
-0.670378702718353));
#15588=CARTESIAN_POINT('Ctrl Pts',(-0.87482617317514,-0.177024326825049,
-0.705826641853758));
#15589=CARTESIAN_POINT('Ctrl Pts',(-0.861652925570091,-0.144299303100741,
-0.721590372101268));
#15590=CARTESIAN_POINT('Ctrl Pts',(-0.848766861100456,-0.0928409665394229,
-0.736604687327351));
#15591=CARTESIAN_POINT('Ctrl Pts',(-0.84559647055299,-0.0762225747374255,
-0.740223768851063));
#15592=CARTESIAN_POINT('Ctrl Pts',(-0.843383895613249,-0.0595300000000001,
-0.742736168477219));
#15593=CARTESIAN_POINT('',(-0.536443649899847,-0.05953,-0.987512846410683));
#15594=CARTESIAN_POINT('Origin',(0.,-0.05953,0.));
#15595=CARTESIAN_POINT('',(0.0548532617164172,-0.05953,-1.12247250791415));
#15596=CARTESIAN_POINT('Ctrl Pts',(-0.536443649899848,-0.0595300000000001,
-0.987512846410683));
#15597=CARTESIAN_POINT('Ctrl Pts',(-0.533501897135712,-0.0762225747374254,
-0.989110885965947));
#15598=CARTESIAN_POINT('Ctrl Pts',(-0.529268075276156,-0.0928409665394227,
-0.991396466802469));
#15599=CARTESIAN_POINT('Ctrl Pts',(-0.511762781179147,-0.144299303100741,
-1.00061845128527));
#15600=CARTESIAN_POINT('Ctrl Pts',(-0.493462957200432,-0.177024326825049,
-1.0099536580922));
#15601=CARTESIAN_POINT('Ctrl Pts',(-0.45280897844858,-0.227269801620063,
-1.02876878445619));
#15602=CARTESIAN_POINT('Ctrl Pts',(-0.425554672694337,-0.251265615809407,
-1.04048957871266));
#15603=CARTESIAN_POINT('Ctrl Pts',(-0.3787731215897,-0.279889827963178,
-1.05829506364875));
#15604=CARTESIAN_POINT('Ctrl Pts',(-0.354166711873529,-0.290879136862659,
-1.06688848765783));
#15605=CARTESIAN_POINT('Ctrl Pts',(-0.302426893214944,-0.305251990234488,
-1.08269251410343));
#15606=CARTESIAN_POINT('Ctrl Pts',(-0.275287440920027,-0.308638795020976,
-1.0898803575765));
#15607=CARTESIAN_POINT('Ctrl Pts',(-0.224855950742601,-0.308638795020976,
-1.10139101611326));
#15608=CARTESIAN_POINT('Ctrl Pts',(-0.19728546073067,-0.305251990234488,
-1.10669035995599));
#15609=CARTESIAN_POINT('Ctrl Pts',(-0.143812384801039,-0.290879136862659,
-1.11490049012186));
#15610=CARTESIAN_POINT('Ctrl Pts',(-0.117914228755037,-0.279889827963178,
-1.1178344036749));
#15611=CARTESIAN_POINT('Ctrl Pts',(-0.0680399972366989,-0.251265615809407,
-1.12208997038458));
#15612=CARTESIAN_POINT('Ctrl Pts',(-0.0383992541984084,-0.227269801620063,
-1.12335509974011));
#15613=CARTESIAN_POINT('Ctrl Pts',(0.00639229239215326,-0.177024326825049,
-1.12404235695137));
#15614=CARTESIAN_POINT('Ctrl Pts',(0.0269302585198977,-0.144299303100741,
-1.12357162229597));
#15615=CARTESIAN_POINT('Ctrl Pts',(0.04670325263426,-0.0928409665394228,
-1.12285816383385));
#15616=CARTESIAN_POINT('Ctrl Pts',(0.0515094706813703,-0.0762225747374255,
-1.12263591311425));
#15617=CARTESIAN_POINT('Ctrl Pts',(0.0548532617164176,-0.0595300000000001,
-1.12247250791414));
#15618=CARTESIAN_POINT('',(0.437601487681057,-0.05953,-1.03511272300331));
#15619=CARTESIAN_POINT('Origin',(0.,-0.05953,0.));
#15620=CARTESIAN_POINT('',(0.911784794170997,-0.05953,-0.656964154625313));
#15621=CARTESIAN_POINT('Ctrl Pts',(0.437601487681056,-0.0595300000000001,
-1.03511272300331));
#15622=CARTESIAN_POINT('Ctrl Pts',(0.440685038163619,-0.0762225747374255,
-1.03380912944435));
#15623=CARTESIAN_POINT('Ctrl Pts',(0.445111721969657,-0.0928409665394228,
-1.03192403056628));
#15624=CARTESIAN_POINT('Ctrl Pts',(0.463236132117164,-0.144299303100741,
-1.0239876538093));
#15625=CARTESIAN_POINT('Ctrl Pts',(0.481944444320713,-0.177024326825049,
-1.01550068154148));
#15626=CARTESIAN_POINT('Ctrl Pts',(0.522002043615455,-0.227269801620064,
-0.995447160474328));
#15627=CARTESIAN_POINT('Ctrl Pts',(0.548158511259203,-0.251265615809407,
-0.981446681891443));
#15628=CARTESIAN_POINT('Ctrl Pts',(0.591247219971725,-0.279889827963178,
-0.955972930713954));
#15629=CARTESIAN_POINT('Ctrl Pts',(0.613307674922609,-0.290879136862659,
-0.942092777160053));
#15630=CARTESIAN_POINT('Ctrl Pts',(0.657923009631182,-0.305251990234487,
-0.91149460735272));
#15631=CARTESIAN_POINT('Ctrl Pts',(0.680463863683393,-0.308638795020976,
-0.894757676234429));
#15632=CARTESIAN_POINT('Ctrl Pts',(0.720906778729542,-0.308638795020976,
-0.862505527716294));
#15633=CARTESIAN_POINT('Ctrl Pts',(0.742239891936899,-0.305251990234488,
-0.844254137480381));
#15634=CARTESIAN_POINT('Ctrl Pts',(0.781998747691872,-0.290879136862659,
-0.80756613568454));
#15635=CARTESIAN_POINT('Ctrl Pts',(0.800439809856112,-0.279889827963178,
-0.789147407129765));
#15636=CARTESIAN_POINT('Ctrl Pts',(0.834863020612702,-0.251265615809407,
-0.752807465209441));
#15637=CARTESIAN_POINT('Ctrl Pts',(0.854332839576145,-0.227269801620064,
-0.73042219438957));
#15638=CARTESIAN_POINT('Ctrl Pts',(0.882797231409153,-0.177024326825049,
-0.695831250979106));
#15639=CARTESIAN_POINT('Ctrl Pts',(0.895234408667242,-0.144299303100741,
-0.679480524217551));
#15640=CARTESIAN_POINT('Ctrl Pts',(0.907004864562642,-0.0928409665394228,
-0.663576540841106));
#15641=CARTESIAN_POINT('Ctrl Pts',(0.909827729890942,-0.0762225747374256,
-0.659680317203144));
#15642=CARTESIAN_POINT('Ctrl Pts',(0.911784794170998,-0.0595300000000001,
-0.656964154625312));
#15643=CARTESIAN_POINT('',(1.08212377959455,-0.05953,-0.303251606722892));
#15644=CARTESIAN_POINT('Origin',(0.,-0.05953,0.));
#15645=CARTESIAN_POINT('',(1.08212377959455,-0.05953,0.303251606722892));
#15646=CARTESIAN_POINT('Ctrl Pts',(1.08212377959455,-0.0595300000000001,
-0.303251606722892));
#15647=CARTESIAN_POINT('Ctrl Pts',(1.0830271513892,-0.0762225747374255,
-0.300028012588062));
#15648=CARTESIAN_POINT('Ctrl Pts',(1.08431331394788,-0.0928409665394228,
-0.2953917518996));
#15649=CARTESIAN_POINT('Ctrl Pts',(1.08940878963422,-0.144299303100741,
-0.276273267473431));
#15650=CARTESIAN_POINT('Ctrl Pts',(1.09443784939331,-0.177024326825049,
-0.256354979351213));
#15651=CARTESIAN_POINT('Ctrl Pts',(1.10373487993589,-0.227269801620064,
-0.212533521233765));
#15652=CARTESIAN_POINT('Ctrl Pts',(1.10909715583869,-0.251265615809407,
-0.183354415742157));
#15653=CARTESIAN_POINT('Ctrl Pts',(1.1160463456491,-0.279889827963178,-0.133783682657561));
#15654=CARTESIAN_POINT('Ctrl Pts',(1.11894887330541,-0.290879136862659,
-0.107881990270302));
#15655=CARTESIAN_POINT('Ctrl Pts',(1.12284346704144,-0.305251990234488,
-0.0539226701638766));
#15656=CARTESIAN_POINT('Ctrl Pts',(1.123812,-0.308638795020976,-0.025864214957475));
#15657=CARTESIAN_POINT('Ctrl Pts',(1.123812,-0.308638795020976,0.025864214957475));
#15658=CARTESIAN_POINT('Ctrl Pts',(1.12284346704144,-0.305251990234488,
0.0539226701638766));
#15659=CARTESIAN_POINT('Ctrl Pts',(1.11894887330541,-0.290879136862659,
0.107881990270302));
#15660=CARTESIAN_POINT('Ctrl Pts',(1.1160463456491,-0.279889827963178,0.133783682657561));
#15661=CARTESIAN_POINT('Ctrl Pts',(1.10909715583869,-0.251265615809407,
0.183354415742157));
#15662=CARTESIAN_POINT('Ctrl Pts',(1.10373487993589,-0.227269801620064,
0.212533521233765));
#15663=CARTESIAN_POINT('Ctrl Pts',(1.09443784939331,-0.177024326825049,
0.256354979351213));
#15664=CARTESIAN_POINT('Ctrl Pts',(1.08940878963422,-0.144299303100741,
0.276273267473431));
#15665=CARTESIAN_POINT('Ctrl Pts',(1.08431331394788,-0.0928409665394228,
0.2953917518996));
#15666=CARTESIAN_POINT('Ctrl Pts',(1.0830271513892,-0.0762225747374255,
0.300028012588062));
#15667=CARTESIAN_POINT('Ctrl Pts',(1.08212377959455,-0.0595300000000001,
0.303251606722892));
#15668=CARTESIAN_POINT('Origin',(0.,-0.05953,0.));
#15669=CARTESIAN_POINT('Origin',(0.,-0.05953,0.));
#15670=CARTESIAN_POINT('',(0.0589974094846122,-0.05953,1.07456964270265));
#15671=CARTESIAN_POINT('Origin',(0.,-0.05953,0.));
#15672=CARTESIAN_POINT('Origin',(-0.244773027351946,-0.05953,1.07242070340001));
#15673=CARTESIAN_POINT('Origin',(-0.244773027351946,0.,1.07242070340001));
#15674=CARTESIAN_POINT('',(-0.519393123750572,-0.05953,0.942555777842682));
#15675=CARTESIAN_POINT('Ctrl Pts',(-0.519393123750572,-0.05953,0.942555777842682));
#15676=CARTESIAN_POINT('Ctrl Pts',(-0.513714466572041,-0.0925528133349865,
0.945684988399766));
#15677=CARTESIAN_POINT('Ctrl Pts',(-0.503136848051455,-0.124911173756694,
0.951483858396181));
#15678=CARTESIAN_POINT('Ctrl Pts',(-0.47593627990192,-0.177924977804098,
0.965323333309091));
#15679=CARTESIAN_POINT('Ctrl Pts',(-0.460931856495794,-0.199697230012983,
0.972669835243841));
#15680=CARTESIAN_POINT('Ctrl Pts',(-0.426157505475872,-0.237895043532788,
0.988400002689705));
#15681=CARTESIAN_POINT('Ctrl Pts',(-0.406380688682952,-0.254319232363049,
0.996771768218699));
#15682=CARTESIAN_POINT('Ctrl Pts',(-0.364750145543744,-0.28018331644634,
1.01272583306292));
#15683=CARTESIAN_POINT('Ctrl Pts',(-0.340838910881557,-0.29104845371857,
1.02112815447116));
#15684=CARTESIAN_POINT('Ctrl Pts',(-0.290495481564827,-0.30527573347708,
1.036574285215));
#15685=CARTESIAN_POINT('Ctrl Pts',(-0.264056468041074,-0.308638795020976,
1.04359501395068));
#15686=CARTESIAN_POINT('Ctrl Pts',(-0.214892249704082,-0.308638795020976,
1.05481642595959));
#15687=CARTESIAN_POINT('Ctrl Pts',(-0.188025341585962,-0.30527573347708,
1.05996242598502));
#15688=CARTESIAN_POINT('Ctrl Pts',(-0.135965654106109,-0.29104845371857,
1.06788913840721));
#15689=CARTESIAN_POINT('Ctrl Pts',(-0.110776745452494,-0.28018331644634,
1.07069360430242));
#15690=CARTESIAN_POINT('Ctrl Pts',(-0.0663467128214646,-0.254319232363049,
1.07438230428002));
#15691=CARTESIAN_POINT('Ctrl Pts',(-0.0448960436540983,-0.237895043532788,
1.07542044338697));
#15692=CARTESIAN_POINT('Ctrl Pts',(-0.00674037211528124,-0.199697230012983,
1.07633607767727));
#15693=CARTESIAN_POINT('Ctrl Pts',(0.00996567398334777,-0.177924977804098,
1.07622728347683));
#15694=CARTESIAN_POINT('Ctrl Pts',(0.0404772621979741,-0.124911173756694,
1.07556023164702));
#15695=CARTESIAN_POINT('Ctrl Pts',(0.0525234025782719,-0.0925528133349865,
1.07492508698591));
#15696=CARTESIAN_POINT('Ctrl Pts',(0.0589974094846124,-0.05953,1.07456964270265));
#15697=CARTESIAN_POINT('Origin',(-0.244773027351946,-0.05953,1.07242070340001));
#15698=CARTESIAN_POINT('Origin',(0.,-0.05953,0.));
#15699=CARTESIAN_POINT('',(-0.803348093619616,-0.05953,0.716109245731214));
#15700=CARTESIAN_POINT('Origin',(0.,-0.05953,0.));
#15701=CARTESIAN_POINT('Origin',(-0.991065754692661,-0.05953,0.477272113029314));
#15702=CARTESIAN_POINT('Origin',(-0.991065754692661,0.,0.477272113029314));
#15703=CARTESIAN_POINT('',(-1.06075609691358,-0.05953,0.181596019242328));
#15704=CARTESIAN_POINT('Ctrl Pts',(-1.06075609691358,-0.05953,0.181596019242328));
#15705=CARTESIAN_POINT('Ctrl Pts',(-1.05966202740332,-0.0925528133349865,
0.187986803072856));
#15706=CARTESIAN_POINT('Ctrl Pts',(-1.05760072925372,-0.124911173756694,
0.199872254546857));
#15707=CARTESIAN_POINT('Ctrl Pts',(-1.05146158959546,-0.177924977804098,
0.22976728653846));
#15708=CARTESIAN_POINT('Ctrl Pts',(-1.04785021111757,-0.199697230012983,
0.246078686169301));
#15709=CARTESIAN_POINT('Ctrl Pts',(-1.03846709802406,-0.237895043532788,
0.283073967563097));
#15710=CARTESIAN_POINT('Ctrl Pts',(-1.03268176429485,-0.254319232363049,
0.303755815985685));
#15711=CARTESIAN_POINT('Ctrl Pts',(-1.01919893537026,-0.28018331644634,
0.346251081972725));
#15712=CARTESIAN_POINT('Ctrl Pts',(-1.01085972381132,-0.29104845371857,
0.370184399726282));
#15713=CARTESIAN_POINT('Ctrl Pts',(-0.99154738033959,-0.30527573347708,
0.419174982698463));
#15714=CARTESIAN_POINT('Ctrl Pts',(-0.980551951791748,-0.308638795020976,
0.444223188605045));
#15715=CARTESIAN_POINT('Ctrl Pts',(-0.958671816228589,-0.308638795020976,
0.489657758261848));
#15716=CARTESIAN_POINT('Ctrl Pts',(-0.945943877838127,-0.30527573347708,
0.51387163140139));
#15717=CARTESIAN_POINT('Ctrl Pts',(-0.91968254693063,-0.29104845371857,
0.559515758398093));
#15718=CARTESIAN_POINT('Ctrl Pts',(-0.906170138993533,-0.28018331644634,
0.580957796077825));
#15719=CARTESIAN_POINT('Ctrl Pts',(-0.8813524085237,-0.254319232363049,
0.617994461173994));
#15720=CARTESIAN_POINT('Ctrl Pts',(-0.868789784891799,-0.237895043532788,
0.635412538795143));
#15721=CARTESIAN_POINT('Ctrl Pts',(-0.845715984518854,-0.199697230012983,
0.66581473268113));
#15722=CARTESIAN_POINT('Ctrl Pts',(-0.835214876415962,-0.177924977804098,
0.678808213394124));
#15723=CARTESIAN_POINT('Ctrl Pts',(-0.815669690204649,-0.124911173756694,
0.702247233627224));
#15724=CARTESIAN_POINT('Ctrl Pts',(-0.807662468433796,-0.0925528133349865,
0.711269279199861));
#15725=CARTESIAN_POINT('Ctrl Pts',(-0.803348093619616,-0.05953,0.716109245731214));
#15726=CARTESIAN_POINT('Origin',(-0.991065754692661,-0.05953,0.477272113029314));
#15727=CARTESIAN_POINT('Origin',(0.,-0.05953,0.));
#15728=CARTESIAN_POINT('',(-1.076188,-0.05953,1.31795018948079E-16));
#15729=CARTESIAN_POINT('Origin',(0.,-0.05953,0.));
#15730=CARTESIAN_POINT('',(-1.06075609691358,-0.05953,-0.181596019242328));
#15731=CARTESIAN_POINT('Origin',(0.,-0.05953,0.));
#15732=CARTESIAN_POINT('Origin',(-0.991065754692661,-0.05953,-0.477272113029314));
#15733=CARTESIAN_POINT('Origin',(-0.991065754692661,0.,-0.477272113029314));
#15734=CARTESIAN_POINT('',(-0.803348093619616,-0.05953,-0.716109245731215));
#15735=CARTESIAN_POINT('Ctrl Pts',(-0.803348093619616,-0.05953,-0.716109245731215));
#15736=CARTESIAN_POINT('Ctrl Pts',(-0.807662468433795,-0.0925528133349865,
-0.711269279199862));
#15737=CARTESIAN_POINT('Ctrl Pts',(-0.815669690204649,-0.124911173756694,
-0.702247233627224));
#15738=CARTESIAN_POINT('Ctrl Pts',(-0.835214876415962,-0.177924977804098,
-0.678808213394124));
#15739=CARTESIAN_POINT('Ctrl Pts',(-0.845715984518854,-0.199697230012983,
-0.66581473268113));
#15740=CARTESIAN_POINT('Ctrl Pts',(-0.868789784891799,-0.237895043532788,
-0.635412538795143));
#15741=CARTESIAN_POINT('Ctrl Pts',(-0.8813524085237,-0.254319232363049,
-0.617994461173994));
#15742=CARTESIAN_POINT('Ctrl Pts',(-0.906170138993533,-0.28018331644634,
-0.580957796077826));
#15743=CARTESIAN_POINT('Ctrl Pts',(-0.91968254693063,-0.29104845371857,
-0.559515758398093));
#15744=CARTESIAN_POINT('Ctrl Pts',(-0.945943877838127,-0.30527573347708,
-0.51387163140139));
#15745=CARTESIAN_POINT('Ctrl Pts',(-0.958671816228589,-0.308638795020976,
-0.489657758261848));
#15746=CARTESIAN_POINT('Ctrl Pts',(-0.980551951791748,-0.308638795020976,
-0.444223188605045));
#15747=CARTESIAN_POINT('Ctrl Pts',(-0.99154738033959,-0.30527573347708,
-0.419174982698463));
#15748=CARTESIAN_POINT('Ctrl Pts',(-1.01085972381132,-0.29104845371857,
-0.370184399726282));
#15749=CARTESIAN_POINT('Ctrl Pts',(-1.01919893537026,-0.28018331644634,
-0.346251081972725));
#15750=CARTESIAN_POINT('Ctrl Pts',(-1.03268176429485,-0.254319232363049,
-0.303755815985685));
#15751=CARTESIAN_POINT('Ctrl Pts',(-1.03846709802406,-0.237895043532788,
-0.283073967563097));
#15752=CARTESIAN_POINT('Ctrl Pts',(-1.04785021111757,-0.199697230012983,
-0.246078686169302));
#15753=CARTESIAN_POINT('Ctrl Pts',(-1.05146158959546,-0.177924977804098,
-0.229767286538461));
#15754=CARTESIAN_POINT('Ctrl Pts',(-1.05760072925372,-0.124911173756694,
-0.199872254546858));
#15755=CARTESIAN_POINT('Ctrl Pts',(-1.05966202740332,-0.0925528133349864,
-0.187986803072857));
#15756=CARTESIAN_POINT('Ctrl Pts',(-1.06075609691358,-0.05953,-0.181596019242328));
#15757=CARTESIAN_POINT('Origin',(-0.991065754692661,-0.05953,-0.477272113029314));
#15758=CARTESIAN_POINT('Origin',(0.,-0.05953,0.));
#15759=CARTESIAN_POINT('',(-0.519393123750572,-0.05953,-0.942555777842682));
#15760=CARTESIAN_POINT('Origin',(0.,-0.05953,0.));
#15761=CARTESIAN_POINT('Origin',(-0.244773027351946,-0.05953,-1.07242070340001));
#15762=CARTESIAN_POINT('Origin',(-0.244773027351946,0.,-1.07242070340001));
#15763=CARTESIAN_POINT('',(0.0589974094846125,-0.05953,-1.07456964270265));
#15764=CARTESIAN_POINT('Ctrl Pts',(0.0589974094846127,-0.05953,-1.07456964270265));
#15765=CARTESIAN_POINT('Ctrl Pts',(0.0525234025782722,-0.0925528133349865,
-1.07492508698591));
#15766=CARTESIAN_POINT('Ctrl Pts',(0.0404772621979744,-0.124911173756694,
-1.07556023164702));
#15767=CARTESIAN_POINT('Ctrl Pts',(0.0099656739833481,-0.177924977804098,
-1.07622728347683));
#15768=CARTESIAN_POINT('Ctrl Pts',(-0.00674037211528096,-0.199697230012983,
-1.07633607767727));
#15769=CARTESIAN_POINT('Ctrl Pts',(-0.044896043654098,-0.237895043532788,
-1.07542044338697));
#15770=CARTESIAN_POINT('Ctrl Pts',(-0.0663467128214644,-0.254319232363049,
-1.07438230428002));
#15771=CARTESIAN_POINT('Ctrl Pts',(-0.110776745452493,-0.28018331644634,
-1.07069360430242));
#15772=CARTESIAN_POINT('Ctrl Pts',(-0.135965654106109,-0.29104845371857,
-1.06788913840721));
#15773=CARTESIAN_POINT('Ctrl Pts',(-0.188025341585962,-0.30527573347708,
-1.05996242598502));
#15774=CARTESIAN_POINT('Ctrl Pts',(-0.214892249704082,-0.308638795020976,
-1.05481642595959));
#15775=CARTESIAN_POINT('Ctrl Pts',(-0.264056468041074,-0.308638795020976,
-1.04359501395068));
#15776=CARTESIAN_POINT('Ctrl Pts',(-0.290495481564827,-0.30527573347708,
-1.036574285215));
#15777=CARTESIAN_POINT('Ctrl Pts',(-0.340838910881557,-0.291048453718569,
-1.02112815447116));
#15778=CARTESIAN_POINT('Ctrl Pts',(-0.364750145543744,-0.28018331644634,
-1.01272583306292));
#15779=CARTESIAN_POINT('Ctrl Pts',(-0.406380688682952,-0.254319232363049,
-0.996771768218699));
#15780=CARTESIAN_POINT('Ctrl Pts',(-0.426157505475872,-0.237895043532788,
-0.988400002689705));
#15781=CARTESIAN_POINT('Ctrl Pts',(-0.460931856495794,-0.199697230012983,
-0.972669835243841));
#15782=CARTESIAN_POINT('Ctrl Pts',(-0.475936279901919,-0.177924977804098,
-0.965323333309091));
#15783=CARTESIAN_POINT('Ctrl Pts',(-0.503136848051454,-0.124911173756694,
-0.951483858396181));
#15784=CARTESIAN_POINT('Ctrl Pts',(-0.513714466572041,-0.0925528133349865,
-0.945684988399766));
#15785=CARTESIAN_POINT('Ctrl Pts',(-0.519393123750572,-0.05953,-0.942555777842682));
#15786=CARTESIAN_POINT('Origin',(-0.244773027351946,-0.05953,-1.07242070340001));
#15787=CARTESIAN_POINT('Origin',(0.,-0.05953,0.));
#15788=CARTESIAN_POINT('',(0.413083465285518,-0.05953,-0.993751811093549));
#15789=CARTESIAN_POINT('Origin',(0.,-0.05953,0.));
#15790=CARTESIAN_POINT('Origin',(0.685838782044607,-0.05953,-0.860014630714833));
#15791=CARTESIAN_POINT('Origin',(0.685838782044607,0.,-0.860014630714833));
#15792=CARTESIAN_POINT('',(0.876916659919095,-0.05953,-0.623857181492959));
#15793=CARTESIAN_POINT('Ctrl Pts',(0.876916659919095,-0.05953,-0.623857181492958));
#15794=CARTESIAN_POINT('Ctrl Pts',(0.873158080166742,-0.0925528133349865,
-0.62914037979579));
#15795=CARTESIAN_POINT('Ctrl Pts',(0.866144010579847,-0.124911173756694,
-0.638954437806245));
#15796=CARTESIAN_POINT('Ctrl Pts',(0.847641868610495,-0.177924977804098,
-0.663225258065736));
#15797=CARTESIAN_POINT('Ctrl Pts',(0.837310877969633,-0.199697230012983,
-0.676354402927683));
#15798=CARTESIAN_POINT('Ctrl Pts',(0.81280533416753,-0.237895043532788,
-0.705614819529209));
#15799=CARTESIAN_POINT('Ctrl Pts',(0.798619410861634,-0.254319232363049,
-0.721738358858166));
#15800=CARTESIAN_POINT('Ctrl Pts',(0.768033796848072,-0.28018331644634,
-0.754175290318038));
#15801=CARTESIAN_POINT('Ctrl Pts',(0.750136149454208,-0.29104845371857,
-0.772120216227122));
#15802=CARTESIAN_POINT('Ctrl Pts',(0.711480111898423,-0.30527573347708,
-0.807879894508811));
#15803=CARTESIAN_POINT('Ctrl Pts',(0.690705563850638,-0.308638795020976,
-0.825676810575913));
#15804=CARTESIAN_POINT('Ctrl Pts',(0.651278921914856,-0.308638795020976,
-0.857118508332695));
#15805=CARTESIAN_POINT('Ctrl Pts',(0.629305439856167,-0.30527573347708,
-0.873412008702649));
#15806=CARTESIAN_POINT('Ctrl Pts',(0.585840553788742,-0.29104845371857,
-0.903141581680914));
#15807=CARTESIAN_POINT('Ctrl Pts',(0.564362943424239,-0.28018331644634,
-0.916597376014514));
#15808=CARTESIAN_POINT('Ctrl Pts',(0.525933334162556,-0.254319232363049,
-0.939198248544427));
#15809=CARTESIAN_POINT('Ctrl Pts',(0.507057380724533,-0.237895043532788,
-0.949440676105255));
#15810=CARTESIAN_POINT('Ctrl Pts',(0.473077587363686,-0.199697230012983,
-0.966820759530997));
#15811=CARTESIAN_POINT('Ctrl Pts',(0.457978755888596,-0.177924977804098,
-0.973971221090534));
#15812=CARTESIAN_POINT('Ctrl Pts',(0.430199341854858,-0.124911173756694,
-0.986608710139579));
#15813=CARTESIAN_POINT('Ctrl Pts',(0.419070565453384,-0.0925528133349865,
-0.991263089003441));
#15814=CARTESIAN_POINT('Ctrl Pts',(0.413083465285518,-0.05953,-0.993751811093549));
#15815=CARTESIAN_POINT('Origin',(0.685838782044607,-0.05953,-0.860014630714833));
#15816=CARTESIAN_POINT('Origin',(0.,-0.208355,0.));
#15817=CARTESIAN_POINT('',(-1.076188,-0.35718,1.31795018948079E-16));
#15818=CARTESIAN_POINT('Origin',(0.,-0.35718,0.));
#15819=CARTESIAN_POINT('',(-1.076188,-0.208355,1.31795018948079E-16));
#15820=CARTESIAN_POINT('',(1.03449977959455,-0.05953,0.296632461748266));
#15821=CARTESIAN_POINT('Origin',(0.,-0.05953,0.));
#15822=CARTESIAN_POINT('',(1.03449977959455,-0.05953,-0.296632461748266));
#15823=CARTESIAN_POINT('Ctrl Pts',(1.03449977959455,-0.05953,0.296632461748267));
#15824=CARTESIAN_POINT('Ctrl Pts',(1.03628691421076,-0.0925528133349865,
0.290399865505497));
#15825=CARTESIAN_POINT('Ctrl Pts',(1.03958665287714,-0.124911173756694,
0.278797079997872));
#15826=CARTESIAN_POINT('Ctrl Pts',(1.0470264474309,-0.177924977804098,0.249198913998601));
#15827=CARTESIAN_POINT('Ctrl Pts',(1.05084995891418,-0.199697230012983,
0.232935932341942));
#15828=CARTESIAN_POINT('Ctrl Pts',(1.05844771715377,-0.237895043532788,
0.195533155353269));
#15829=CARTESIAN_POINT('Ctrl Pts',(1.06220882929878,-0.254319232363049,
0.17438929156337));
#15830=CARTESIAN_POINT('Ctrl Pts',(1.06849922508772,-0.28018331644634,0.130252399648131));
#15831=CARTESIAN_POINT('Ctrl Pts',(1.07137013248666,-0.29104845371857,0.105070977154072));
#15832=CARTESIAN_POINT('Ctrl Pts',(1.07522652957392,-0.30527573347708,0.0525526752791107));
#15833=CARTESIAN_POINT('Ctrl Pts',(1.076188,-0.308638795020976,0.025214283908933));
#15834=CARTESIAN_POINT('Ctrl Pts',(1.076188,-0.308638795020976,-0.025214283908933));
#15835=CARTESIAN_POINT('Ctrl Pts',(1.07522652957392,-0.30527573347708,-0.0525526752791107));
#15836=CARTESIAN_POINT('Ctrl Pts',(1.07137013248666,-0.29104845371857,-0.105070977154072));
#15837=CARTESIAN_POINT('Ctrl Pts',(1.06849922508772,-0.28018331644634,-0.130252399648131));
#15838=CARTESIAN_POINT('Ctrl Pts',(1.06220882929878,-0.254319232363049,
-0.17438929156337));
#15839=CARTESIAN_POINT('Ctrl Pts',(1.05844771715377,-0.237895043532788,
-0.195533155353269));
#15840=CARTESIAN_POINT('Ctrl Pts',(1.05084995891418,-0.199697230012983,
-0.232935932341942));
#15841=CARTESIAN_POINT('Ctrl Pts',(1.0470264474309,-0.177924977804098,-0.249198913998601));
#15842=CARTESIAN_POINT('Ctrl Pts',(1.03958665287714,-0.124911173756694,
-0.278797079997872));
#15843=CARTESIAN_POINT('Ctrl Pts',(1.03628691421076,-0.0925528133349865,
-0.290399865505497));
#15844=CARTESIAN_POINT('Ctrl Pts',(1.03449977959455,-0.05953,-0.296632461748267));
#15845=CARTESIAN_POINT('Origin',(0.,-0.05953,0.));
#15846=CARTESIAN_POINT('Origin',(0.,-0.05953,0.));
#15847=CARTESIAN_POINT('Origin',(1.1,-0.05953,0.));
#15848=CARTESIAN_POINT('Origin',(1.1,0.,0.));
#15849=CARTESIAN_POINT('Origin',(1.1,-0.05953,0.));
#15850=CARTESIAN_POINT('Origin',(0.,-0.35718,0.));
#15851=CARTESIAN_POINT('Origin',(0.,-0.05953,0.));
#17760=UNCERTAINTY_MEASURE_WITH_UNIT(LENGTH_MEASURE(0.001),#17831,
'DISTANCE_ACCURACY_VALUE',
'Maximum model space distance between geometric entities at asserted c
onnectivities');
#17780=UNCERTAINTY_MEASURE_WITH_UNIT(LENGTH_MEASURE(0.001),#17831,
'DISTANCE_ACCURACY_VALUE',
'Maximum model space distance between geometric entities at asserted c
onnectivities');
#17810=(
GEOMETRIC_REPRESENTATION_CONTEXT(3)
GLOBAL_UNCERTAINTY_ASSIGNED_CONTEXT((#17760))
GLOBAL_UNIT_ASSIGNED_CONTEXT((#17831,#17833,#17834))
REPRESENTATION_CONTEXT('','3D')
);
#17830=(
GEOMETRIC_REPRESENTATION_CONTEXT(3)
GLOBAL_UNCERTAINTY_ASSIGNED_CONTEXT((#17780))
GLOBAL_UNIT_ASSIGNED_CONTEXT((#17831,#17833,#17834))
REPRESENTATION_CONTEXT('','3D')
);
#17831=(
LENGTH_UNIT()
NAMED_UNIT(*)
SI_UNIT(.CENTI.,.METRE.)
);
#17833=(
NAMED_UNIT(*)
PLANE_ANGLE_UNIT()
SI_UNIT($,.RADIAN.)
);
#17834=(
NAMED_UNIT(*)
SI_UNIT($,.STERADIAN.)
SOLID_ANGLE_UNIT()
);
#17864=SHAPE_DEFINITION_REPRESENTATION(#17918,#18035);
#17918=PRODUCT_DEFINITION_SHAPE('',$,#18085);
#18035=SHAPE_REPRESENTATION('',(#10096),#17810);
#18055=PRODUCT_DEFINITION_CONTEXT('part definition',#18204,'design');
#18085=PRODUCT_DEFINITION('Cage (1)','Cage (1)',#18134,#18055);
#18134=PRODUCT_DEFINITION_FORMATION('',$,#18235);
#18204=APPLICATION_CONTEXT(
'Core Data for Automotive Mechanical Design Process');
#18205=PRODUCT_CONTEXT('part definition',#18204,'mechanical');
#18235=PRODUCT('Cage (1)','Cage (1)','Cage (1)',(#18205));
#18311=COLOUR_RGB('Grey',0.48,0.52,0.57);
#18312=FILL_AREA_STYLE_COLOUR('',#18311);
#18313=FILL_AREA_STYLE('',(#18312));
#18314=SURFACE_STYLE_FILL_AREA(#18313);
#18315=SURFACE_SIDE_STYLE('',(#18314));
#18316=SURFACE_STYLE_USAGE(.BOTH.,#18315);
#18317=PRESENTATION_STYLE_ASSIGNMENT((#18316));
ENDSEC;
END-ISO-10303-21;
